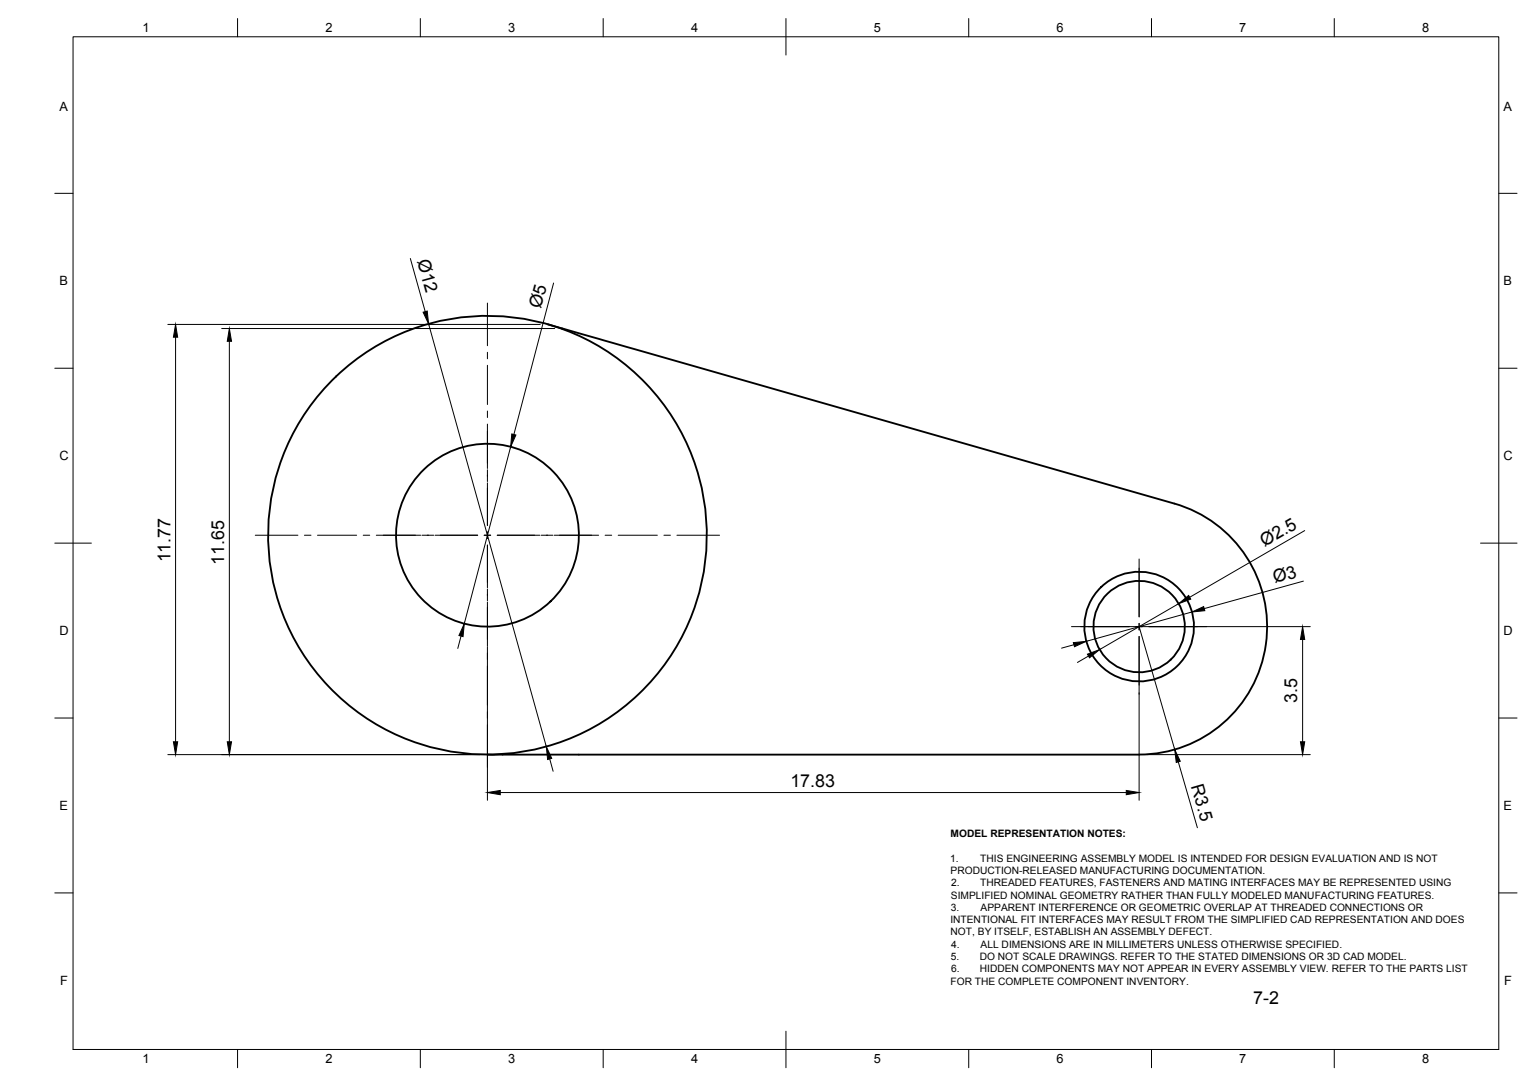
ISO-10303-21;
HEADER;
/* Generated by software containing ST-Developer
 * from STEP Tools, Inc. (www.steptools.com) 
 */

FILE_DESCRIPTION(
/* description */ (''),
/* implementation_level */ '2;1');

FILE_NAME(
/* name */ '7-2.step',
/* time_stamp */ '2026-10-06T01:16:10-07:00',
/* author */ (''),
/* organization */ (''),
/* preprocessor_version */ 'ST-DEVELOPER v20.2',
/* originating_system */ 'Autodesk Translation Framework v15.15.0.0',
/* authorisation */ '');

FILE_SCHEMA (('AUTOMOTIVE_DESIGN { 1 0 10303 214 3 1 1 }'));
ENDSEC;

DATA;
#10=MECHANICAL_DESIGN_GEOMETRIC_PRESENTATION_REPRESENTATION('',(#307,#308),#17113);
#107=ELLIPSE('',#6627,1.26223360526973,1.25);
#108=ELLIPSE('',#6640,1.26223360526973,1.25);
#135=TOROIDAL_SURFACE('',#6625,6.5,0.5);
#136=TOROIDAL_SURFACE('',#6631,5.7,0.3);
#137=TOROIDAL_SURFACE('',#6636,3.2,0.3);
#176=B_SPLINE_CURVE_WITH_KNOTS('',3,(#10699,#10700,#10701,#10702,#10703,
#10704,#10705,#10706,#10707,#10708),.UNSPECIFIED.,.F.,.F.,(4,2,2,2,4),(-0.377880095159423,
-0.330643519967439,-0.283406944775455,-0.236173496177583,-0.188940047579712),
 .UNSPECIFIED.);
#177=B_SPLINE_CURVE_WITH_KNOTS('',3,(#10712,#10713,#10714,#10715,#10716,
#10717,#10718,#10719,#10720,#10721),.UNSPECIFIED.,.F.,.F.,(4,2,2,2,4),(0.188940047579712,
0.236173496177583,0.283406944775455,0.330643519967439,0.377880095159423),
 .UNSPECIFIED.);
#178=B_SPLINE_CURVE_WITH_KNOTS('',3,(#10723,#10724,#10725,#10726,#10727,
#10728,#10729,#10730,#10731,#10732,#10733,#10734,#10735,#10736,#10737,#10738,
#10739,#10740,#10741,#10742,#10743,#10744,#10745),.UNSPECIFIED.,.F.,.F.,
(4,2,2,2,2,2,3,2,2,2,4),(-0.276474823920439,-0.236173496177583,-0.188940047579712,
-0.14170659898184,-0.0944731503839682,-0.0472365751919841,0.,0.0472365751919841,
0.0944731503839681,0.14170659898184,0.188940047579712),.UNSPECIFIED.);
#179=B_SPLINE_CURVE_WITH_KNOTS('',3,(#10752,#10753,#10754,#10755,#10756,
#10757,#10758,#10759,#10760,#10761,#10762,#10763,#10764,#10765,#10766,#10767,
#10768,#10769,#10770),.UNSPECIFIED.,.F.,.F.,(4,2,2,2,3,2,2,2,4),(-0.188940047579712,
-0.14170659898184,-0.0944731503839681,-0.0472365751919841,0.,0.0472365751919841,
0.0944731503839682,0.14170659898184,0.188940047579712),.UNSPECIFIED.);
#180=B_SPLINE_CURVE_WITH_KNOTS('',3,(#10799,#10800,#10801,#10802),
 .UNSPECIFIED.,.F.,.F.,(4,4),(0.0419009061515246,0.24114214195851),
 .UNSPECIFIED.);
#181=B_SPLINE_CURVE_WITH_KNOTS('',3,(#10803,#10804,#10805,#10806,#10807,
#10808),.UNSPECIFIED.,.F.,.F.,(4,2,4),(-0.160890299009028,-0.155410119436095,
-0.148763314259543),.UNSPECIFIED.);
#182=B_SPLINE_CURVE_WITH_KNOTS('',3,(#10810,#10811,#10812,#10813,#10814,
#10815),.UNSPECIFIED.,.F.,.F.,(4,2,4),(-0.173042755318085,-0.172254926856018,
-0.160890299013474),.UNSPECIFIED.);
#183=B_SPLINE_CURVE_WITH_KNOTS('',3,(#10816,#10817,#10818,#10819),
 .UNSPECIFIED.,.F.,.F.,(4,4),(0.488884303449535,0.688125539256493),
 .UNSPECIFIED.);
#184=B_SPLINE_CURVE_WITH_KNOTS('',3,(#10845,#10846,#10847,#10848,#10849,
#10850),.UNSPECIFIED.,.F.,.F.,(4,2,4),(0.188940047579712,0.236173496177584,
0.276474823920109),.UNSPECIFIED.);
#185=B_SPLINE_CURVE_WITH_KNOTS('',3,(#10854,#10855,#10856,#10857,#10858,
#10859,#10860,#10861,#10862,#10863,#10864,#10865,#10866,#10867,#10868,#10869,
#10870,#10871),.UNSPECIFIED.,.F.,.F.,(4,2,2,2,2,2,2,2,4),(0.192195276051885,
0.240178513967644,0.288161751883402,0.336276151993586,0.38439055210377,
0.432504952213954,0.480619352324138,0.528602590239897,0.576585828155655),
 .UNSPECIFIED.);
#186=B_SPLINE_CURVE_WITH_KNOTS('',3,(#10872,#10873,#10874,#10875,#10876,
#10877,#10878,#10879,#10880,#10881,#10882,#10883,#10884,#10885,#10886,#10887,
#10888,#10889,#10890),.UNSPECIFIED.,.F.,.F.,(4,2,2,2,3,2,2,2,4),(-0.192195276051885,
-0.144212038136127,-0.0962288002203683,-0.0481144001101841,1.11022302462516E-16,
0.0481144001101843,0.0962288002203684,0.144212038136127,0.192195276051885),
 .UNSPECIFIED.);
#187=B_SPLINE_CURVE_WITH_KNOTS('',3,(#10894,#10895,#10896,#10897,#10898,
#10899,#10900,#10901,#10902,#10903,#10904,#10905,#10906,#10907,#10908,#10909,
#10910,#10911,#10912),.UNSPECIFIED.,.F.,.F.,(4,2,2,2,3,2,2,2,4),(-0.192195276051885,
-0.144212038136127,-0.0962288002203683,-0.0481144001101841,0.,0.0481144001101841,
0.0962288002203683,0.144212038136127,0.192195276051885),.UNSPECIFIED.);
#188=B_SPLINE_CURVE_WITH_KNOTS('',3,(#10913,#10914,#10915,#10916,#10917,
#10918,#10919,#10920,#10921,#10922,#10923,#10924,#10925,#10926,#10927,#10928,
#10929,#10930),.UNSPECIFIED.,.F.,.F.,(4,2,2,2,2,2,2,2,4),(0.192195276051885,
0.240178513967643,0.288161751883402,0.336276151993586,0.38439055210377,
0.432504952213954,0.480619352324138,0.528602590239897,0.576585828155655),
 .UNSPECIFIED.);
#227=OPEN_SHELL('',(#5864,#5865));
#245=SHELL_BASED_SURFACE_MODEL('Body2',(#227));
#269=SHAPE_REPRESENTATION_RELATIONSHIP('SRR','None',#17193,#285);
#285=ADVANCED_BREP_SHAPE_REPRESENTATION('',(#335),#17100);
#307=STYLED_ITEM('',(#17298),#335);
#308=STYLED_ITEM('',(#17298),#245);
#335=MANIFOLD_SOLID_BREP('Body1',#6021);
#431=CYLINDRICAL_SURFACE('',#6611,6.);
#432=CYLINDRICAL_SURFACE('',#6620,1.25);
#433=CYLINDRICAL_SURFACE('',#6628,0.3);
#434=CYLINDRICAL_SURFACE('',#6634,0.3);
#435=CYLINDRICAL_SURFACE('',#6638,3.5);
#436=CYLINDRICAL_SURFACE('',#6641,1.25);
#437=CYLINDRICAL_SURFACE('',#6642,1.25);
#438=CYLINDRICAL_SURFACE('',#6643,6.);
#439=CYLINDRICAL_SURFACE('',#6644,2.5);
#440=CYLINDRICAL_SURFACE('',#6647,1.5);
#577=FACE_BOUND('',#1634,.T.);
#578=FACE_BOUND('',#1635,.T.);
#579=FACE_BOUND('',#1638,.T.);
#580=FACE_BOUND('',#1651,.T.);
#581=FACE_BOUND('',#1653,.T.);
#582=FACE_BOUND('',#1656,.T.);
#836=CIRCLE('',#6612,6.);
#837=CIRCLE('',#6613,6.);
#838=CIRCLE('',#6614,6.);
#839=CIRCLE('',#6616,5.7);
#840=CIRCLE('',#6617,3.2);
#841=CIRCLE('',#6618,2.5);
#842=CIRCLE('',#6619,1.25);
#843=CIRCLE('',#6621,1.25);
#844=CIRCLE('',#6623,6.5);
#845=CIRCLE('',#6624,3.5);
#846=CIRCLE('',#6629,0.3);
#847=CIRCLE('',#6630,0.3);
#848=CIRCLE('',#6632,6.);
#849=CIRCLE('',#6633,0.3);
#850=CIRCLE('',#6635,0.3);
#851=CIRCLE('',#6637,3.5);
#852=CIRCLE('',#6645,2.5);
#853=CIRCLE('',#6648,1.5);
#854=CIRCLE('',#6649,1.5);
#855=CIRCLE('',#6651,1.25);
#1199=FACE_OUTER_BOUND('',#1632,.T.);
#1200=FACE_OUTER_BOUND('',#1633,.T.);
#1201=FACE_OUTER_BOUND('',#1636,.T.);
#1202=FACE_OUTER_BOUND('',#1637,.T.);
#1203=FACE_OUTER_BOUND('',#1639,.T.);
#1204=FACE_OUTER_BOUND('',#1640,.T.);
#1205=FACE_OUTER_BOUND('',#1641,.T.);
#1206=FACE_OUTER_BOUND('',#1642,.T.);
#1207=FACE_OUTER_BOUND('',#1643,.T.);
#1208=FACE_OUTER_BOUND('',#1644,.T.);
#1209=FACE_OUTER_BOUND('',#1645,.T.);
#1210=FACE_OUTER_BOUND('',#1646,.T.);
#1211=FACE_OUTER_BOUND('',#1647,.T.);
#1212=FACE_OUTER_BOUND('',#1648,.T.);
#1213=FACE_OUTER_BOUND('',#1649,.T.);
#1214=FACE_OUTER_BOUND('',#1650,.T.);
#1215=FACE_OUTER_BOUND('',#1652,.T.);
#1216=FACE_OUTER_BOUND('',#1654,.T.);
#1217=FACE_OUTER_BOUND('',#1655,.T.);
#1632=EDGE_LOOP('',(#4788,#4789,#4790,#4791,#4792,#4793,#4794,#4795,#4796,
#4797,#4798));
#1633=EDGE_LOOP('',(#4799,#4800,#4801,#4802));
#1634=EDGE_LOOP('',(#4803));
#1635=EDGE_LOOP('',(#4804));
#1636=EDGE_LOOP('',(#4805,#4806,#4807,#4808));
#1637=EDGE_LOOP('',(#4809,#4810,#4811,#4812));
#1638=EDGE_LOOP('',(#4813));
#1639=EDGE_LOOP('',(#4814,#4815,#4816,#4817,#4818,#4819));
#1640=EDGE_LOOP('',(#4820,#4821,#4822,#4823,#4824,#4825));
#1641=EDGE_LOOP('',(#4826,#4827,#4828,#4829));
#1642=EDGE_LOOP('',(#4830,#4831,#4832,#4833,#4834));
#1643=EDGE_LOOP('',(#4835,#4836,#4837,#4838));
#1644=EDGE_LOOP('',(#4839,#4840,#4841,#4842));
#1645=EDGE_LOOP('',(#4843,#4844,#4845,#4846));
#1646=EDGE_LOOP('',(#4847,#4848,#4849,#4850,#4851,#4852));
#1647=EDGE_LOOP('',(#4853,#4854,#4855,#4856,#4857,#4858,#4859,#4860,#4861));
#1648=EDGE_LOOP('',(#4862,#4863,#4864,#4865,#4866,#4867,#4868,#4869));
#1649=EDGE_LOOP('',(#4870,#4871,#4872,#4873));
#1650=EDGE_LOOP('',(#4874,#4875,#4876,#4877,#4878,#4879,#4880,#4881));
#1651=EDGE_LOOP('',(#4882,#4883));
#1652=EDGE_LOOP('',(#4884));
#1653=EDGE_LOOP('',(#4885));
#1654=EDGE_LOOP('',(#4886,#4887,#4888,#4889));
#1655=EDGE_LOOP('',(#4890));
#1656=EDGE_LOOP('',(#4891));
#2070=LINE('',#10697,#2431);
#2071=LINE('',#10747,#2432);
#2072=LINE('',#10751,#2433);
#2073=LINE('',#10776,#2434);
#2074=LINE('',#10779,#2435);
#2075=LINE('',#10786,#2436);
#2076=LINE('',#10793,#2437);
#2077=LINE('',#10796,#2438);
#2078=LINE('',#10823,#2439);
#2079=LINE('',#10824,#2440);
#2080=LINE('',#10827,#2441);
#2081=LINE('',#10836,#2442);
#2082=LINE('',#10841,#2443);
#2083=LINE('',#10852,#2444);
#2084=LINE('',#10931,#2445);
#2085=LINE('',#10934,#2446);
#2086=LINE('',#10936,#2447);
#2087=LINE('',#10943,#2448);
#2431=VECTOR('',#7996,6.);
#2432=VECTOR('',#7999,3.268305009375);
#2433=VECTOR('',#8002,6.);
#2434=VECTOR('',#8007,17.82554346998);
#2435=VECTOR('',#8010,17.8255434699797);
#2436=VECTOR('',#8017,1.25);
#2437=VECTOR('',#8024,15.3255434699798);
#2438=VECTOR('',#8027,15.3255434699798);
#2439=VECTOR('',#8032,17.8255434887197);
#2440=VECTOR('',#8033,3.7);
#2441=VECTOR('',#8036,3.268305009375);
#2442=VECTOR('',#8051,17.8255434620497);
#2443=VECTOR('',#8060,3.7);
#2444=VECTOR('',#8067,1.25);
#2445=VECTOR('',#8070,1.25);
#2446=VECTOR('',#8075,2.5);
#2447=VECTOR('',#8076,2.5);
#2448=VECTOR('',#8085,1.5);
#2858=VERTEX_POINT('',#10694);
#2859=VERTEX_POINT('',#10696);
#2860=VERTEX_POINT('',#10698);
#2861=VERTEX_POINT('',#10709);
#2862=VERTEX_POINT('',#10711);
#2863=VERTEX_POINT('',#10722);
#2864=VERTEX_POINT('',#10746);
#2865=VERTEX_POINT('',#10748);
#2866=VERTEX_POINT('',#10750);
#2867=VERTEX_POINT('',#10772);
#2868=VERTEX_POINT('',#10773);
#2869=VERTEX_POINT('',#10775);
#2870=VERTEX_POINT('',#10777);
#2871=VERTEX_POINT('',#10780);
#2872=VERTEX_POINT('',#10782);
#2873=VERTEX_POINT('',#10785);
#2874=VERTEX_POINT('',#10789);
#2875=VERTEX_POINT('',#10790);
#2876=VERTEX_POINT('',#10792);
#2877=VERTEX_POINT('',#10794);
#2878=VERTEX_POINT('',#10798);
#2879=VERTEX_POINT('',#10809);
#2880=VERTEX_POINT('',#10821);
#2881=VERTEX_POINT('',#10822);
#2882=VERTEX_POINT('',#10825);
#2883=VERTEX_POINT('',#10835);
#2884=VERTEX_POINT('',#10851);
#2885=VERTEX_POINT('',#10853);
#2886=VERTEX_POINT('',#10892);
#2887=VERTEX_POINT('',#10893);
#2888=VERTEX_POINT('',#10935);
#2889=VERTEX_POINT('',#10940);
#2890=VERTEX_POINT('',#10942);
#2891=VERTEX_POINT('',#10946);
#3546=EDGE_CURVE('',#2858,#2858,#836,.T.);
#3547=EDGE_CURVE('',#2858,#2859,#2070,.T.);
#3548=EDGE_CURVE('',#2859,#2860,#176,.F.);
#3549=EDGE_CURVE('',#2860,#2861,#837,.T.);
#3550=EDGE_CURVE('',#2861,#2862,#177,.F.);
#3551=EDGE_CURVE('',#2862,#2863,#178,.F.);
#3552=EDGE_CURVE('',#2864,#2863,#2071,.T.);
#3553=EDGE_CURVE('',#2865,#2864,#838,.T.);
#3554=EDGE_CURVE('',#2866,#2865,#2072,.T.);
#3555=EDGE_CURVE('',#2866,#2859,#179,.F.);
#3556=EDGE_CURVE('',#2867,#2868,#839,.T.);
#3557=EDGE_CURVE('',#2868,#2869,#2073,.T.);
#3558=EDGE_CURVE('',#2869,#2870,#840,.T.);
#3559=EDGE_CURVE('',#2870,#2867,#2074,.T.);
#3560=EDGE_CURVE('',#2871,#2871,#841,.T.);
#3561=EDGE_CURVE('',#2872,#2872,#842,.T.);
#3562=EDGE_CURVE('',#2872,#2873,#2075,.T.);
#3563=EDGE_CURVE('',#2873,#2873,#843,.T.);
#3564=EDGE_CURVE('',#2874,#2875,#844,.T.);
#3565=EDGE_CURVE('',#2874,#2876,#2076,.T.);
#3566=EDGE_CURVE('',#2876,#2877,#845,.T.);
#3567=EDGE_CURVE('',#2877,#2875,#2077,.T.);
#3568=EDGE_CURVE('',#2878,#2875,#180,.T.);
#3569=EDGE_CURVE('',#2861,#2878,#181,.T.);
#3570=EDGE_CURVE('',#2879,#2860,#182,.T.);
#3571=EDGE_CURVE('',#2874,#2879,#183,.T.);
#3572=EDGE_CURVE('',#2880,#2881,#2078,.T.);
#3573=EDGE_CURVE('',#2880,#2876,#2079,.T.);
#3574=EDGE_CURVE('',#2879,#2882,#107,.T.);
#3575=EDGE_CURVE('',#2881,#2882,#2080,.T.);
#3576=EDGE_CURVE('',#2870,#2880,#846,.T.);
#3577=EDGE_CURVE('',#2867,#2881,#847,.T.);
#3578=EDGE_CURVE('',#2881,#2865,#848,.T.);
#3579=EDGE_CURVE('',#2868,#2864,#849,.T.);
#3580=EDGE_CURVE('',#2864,#2883,#2081,.T.);
#3581=EDGE_CURVE('',#2869,#2883,#850,.T.);
#3582=EDGE_CURVE('',#2883,#2880,#851,.T.);
#3583=EDGE_CURVE('',#2883,#2877,#2082,.T.);
#3584=EDGE_CURVE('',#2878,#2863,#108,.T.);
#3585=EDGE_CURVE('',#2882,#2866,#184,.F.);
#3586=EDGE_CURVE('',#2859,#2884,#2083,.T.);
#3587=EDGE_CURVE('',#2885,#2884,#185,.T.);
#3588=EDGE_CURVE('',#2884,#2885,#186,.T.);
#3589=EDGE_CURVE('',#2886,#2887,#187,.T.);
#3590=EDGE_CURVE('',#2887,#2886,#188,.T.);
#3591=EDGE_CURVE('',#2887,#2862,#2084,.T.);
#3592=EDGE_CURVE('',#2871,#2885,#2085,.T.);
#3593=EDGE_CURVE('',#2884,#2888,#2086,.T.);
#3594=EDGE_CURVE('',#2888,#2888,#852,.T.);
#3595=EDGE_CURVE('',#2889,#2889,#853,.T.);
#3596=EDGE_CURVE('',#2889,#2890,#2087,.T.);
#3597=EDGE_CURVE('',#2890,#2890,#854,.T.);
#3598=EDGE_CURVE('',#2891,#2891,#855,.T.);
#4788=ORIENTED_EDGE('',*,*,#3546,.F.);
#4789=ORIENTED_EDGE('',*,*,#3547,.T.);
#4790=ORIENTED_EDGE('',*,*,#3548,.T.);
#4791=ORIENTED_EDGE('',*,*,#3549,.T.);
#4792=ORIENTED_EDGE('',*,*,#3550,.T.);
#4793=ORIENTED_EDGE('',*,*,#3551,.T.);
#4794=ORIENTED_EDGE('',*,*,#3552,.F.);
#4795=ORIENTED_EDGE('',*,*,#3553,.F.);
#4796=ORIENTED_EDGE('',*,*,#3554,.F.);
#4797=ORIENTED_EDGE('',*,*,#3555,.T.);
#4798=ORIENTED_EDGE('',*,*,#3547,.F.);
#4799=ORIENTED_EDGE('',*,*,#3556,.T.);
#4800=ORIENTED_EDGE('',*,*,#3557,.T.);
#4801=ORIENTED_EDGE('',*,*,#3558,.T.);
#4802=ORIENTED_EDGE('',*,*,#3559,.T.);
#4803=ORIENTED_EDGE('',*,*,#3560,.F.);
#4804=ORIENTED_EDGE('',*,*,#3561,.F.);
#4805=ORIENTED_EDGE('',*,*,#3561,.T.);
#4806=ORIENTED_EDGE('',*,*,#3562,.T.);
#4807=ORIENTED_EDGE('',*,*,#3563,.F.);
#4808=ORIENTED_EDGE('',*,*,#3562,.F.);
#4809=ORIENTED_EDGE('',*,*,#3564,.F.);
#4810=ORIENTED_EDGE('',*,*,#3565,.T.);
#4811=ORIENTED_EDGE('',*,*,#3566,.T.);
#4812=ORIENTED_EDGE('',*,*,#3567,.T.);
#4813=ORIENTED_EDGE('',*,*,#3563,.T.);
#4814=ORIENTED_EDGE('',*,*,#3564,.T.);
#4815=ORIENTED_EDGE('',*,*,#3568,.F.);
#4816=ORIENTED_EDGE('',*,*,#3569,.F.);
#4817=ORIENTED_EDGE('',*,*,#3549,.F.);
#4818=ORIENTED_EDGE('',*,*,#3570,.F.);
#4819=ORIENTED_EDGE('',*,*,#3571,.F.);
#4820=ORIENTED_EDGE('',*,*,#3572,.F.);
#4821=ORIENTED_EDGE('',*,*,#3573,.T.);
#4822=ORIENTED_EDGE('',*,*,#3565,.F.);
#4823=ORIENTED_EDGE('',*,*,#3571,.T.);
#4824=ORIENTED_EDGE('',*,*,#3574,.T.);
#4825=ORIENTED_EDGE('',*,*,#3575,.F.);
#4826=ORIENTED_EDGE('',*,*,#3559,.F.);
#4827=ORIENTED_EDGE('',*,*,#3576,.T.);
#4828=ORIENTED_EDGE('',*,*,#3572,.T.);
#4829=ORIENTED_EDGE('',*,*,#3577,.F.);
#4830=ORIENTED_EDGE('',*,*,#3556,.F.);
#4831=ORIENTED_EDGE('',*,*,#3577,.T.);
#4832=ORIENTED_EDGE('',*,*,#3578,.T.);
#4833=ORIENTED_EDGE('',*,*,#3553,.T.);
#4834=ORIENTED_EDGE('',*,*,#3579,.F.);
#4835=ORIENTED_EDGE('',*,*,#3557,.F.);
#4836=ORIENTED_EDGE('',*,*,#3579,.T.);
#4837=ORIENTED_EDGE('',*,*,#3580,.T.);
#4838=ORIENTED_EDGE('',*,*,#3581,.F.);
#4839=ORIENTED_EDGE('',*,*,#3558,.F.);
#4840=ORIENTED_EDGE('',*,*,#3581,.T.);
#4841=ORIENTED_EDGE('',*,*,#3582,.T.);
#4842=ORIENTED_EDGE('',*,*,#3576,.F.);
#4843=ORIENTED_EDGE('',*,*,#3582,.F.);
#4844=ORIENTED_EDGE('',*,*,#3583,.T.);
#4845=ORIENTED_EDGE('',*,*,#3566,.F.);
#4846=ORIENTED_EDGE('',*,*,#3573,.F.);
#4847=ORIENTED_EDGE('',*,*,#3580,.F.);
#4848=ORIENTED_EDGE('',*,*,#3552,.T.);
#4849=ORIENTED_EDGE('',*,*,#3584,.F.);
#4850=ORIENTED_EDGE('',*,*,#3568,.T.);
#4851=ORIENTED_EDGE('',*,*,#3567,.F.);
#4852=ORIENTED_EDGE('',*,*,#3583,.F.);
#4853=ORIENTED_EDGE('',*,*,#3585,.F.);
#4854=ORIENTED_EDGE('',*,*,#3574,.F.);
#4855=ORIENTED_EDGE('',*,*,#3570,.T.);
#4856=ORIENTED_EDGE('',*,*,#3548,.F.);
#4857=ORIENTED_EDGE('',*,*,#3586,.T.);
#4858=ORIENTED_EDGE('',*,*,#3587,.F.);
#4859=ORIENTED_EDGE('',*,*,#3588,.F.);
#4860=ORIENTED_EDGE('',*,*,#3586,.F.);
#4861=ORIENTED_EDGE('',*,*,#3555,.F.);
#4862=ORIENTED_EDGE('',*,*,#3589,.F.);
#4863=ORIENTED_EDGE('',*,*,#3590,.F.);
#4864=ORIENTED_EDGE('',*,*,#3591,.T.);
#4865=ORIENTED_EDGE('',*,*,#3550,.F.);
#4866=ORIENTED_EDGE('',*,*,#3569,.T.);
#4867=ORIENTED_EDGE('',*,*,#3584,.T.);
#4868=ORIENTED_EDGE('',*,*,#3551,.F.);
#4869=ORIENTED_EDGE('',*,*,#3591,.F.);
#4870=ORIENTED_EDGE('',*,*,#3554,.T.);
#4871=ORIENTED_EDGE('',*,*,#3578,.F.);
#4872=ORIENTED_EDGE('',*,*,#3575,.T.);
#4873=ORIENTED_EDGE('',*,*,#3585,.T.);
#4874=ORIENTED_EDGE('',*,*,#3560,.T.);
#4875=ORIENTED_EDGE('',*,*,#3592,.T.);
#4876=ORIENTED_EDGE('',*,*,#3587,.T.);
#4877=ORIENTED_EDGE('',*,*,#3593,.T.);
#4878=ORIENTED_EDGE('',*,*,#3594,.F.);
#4879=ORIENTED_EDGE('',*,*,#3593,.F.);
#4880=ORIENTED_EDGE('',*,*,#3588,.T.);
#4881=ORIENTED_EDGE('',*,*,#3592,.F.);
#4882=ORIENTED_EDGE('',*,*,#3589,.T.);
#4883=ORIENTED_EDGE('',*,*,#3590,.T.);
#4884=ORIENTED_EDGE('',*,*,#3546,.T.);
#4885=ORIENTED_EDGE('',*,*,#3594,.T.);
#4886=ORIENTED_EDGE('',*,*,#3595,.F.);
#4887=ORIENTED_EDGE('',*,*,#3596,.T.);
#4888=ORIENTED_EDGE('',*,*,#3597,.T.);
#4889=ORIENTED_EDGE('',*,*,#3596,.F.);
#4890=ORIENTED_EDGE('',*,*,#3597,.F.);
#4891=ORIENTED_EDGE('',*,*,#3598,.F.);
#5577=PLANE('',#6615);
#5578=PLANE('',#6622);
#5579=PLANE('',#6626);
#5580=PLANE('',#6639);
#5581=PLANE('',#6646);
#5582=PLANE('',#6650);
#5847=ADVANCED_FACE('',(#1199),#431,.T.);
#5848=ADVANCED_FACE('',(#1200,#577,#578),#5577,.F.);
#5849=ADVANCED_FACE('',(#1201),#432,.F.);
#5850=ADVANCED_FACE('',(#1202,#579),#5578,.T.);
#5851=ADVANCED_FACE('',(#1203),#135,.F.);
#5852=ADVANCED_FACE('',(#1204),#5579,.T.);
#5853=ADVANCED_FACE('',(#1205),#433,.T.);
#5854=ADVANCED_FACE('',(#1206),#136,.T.);
#5855=ADVANCED_FACE('',(#1207),#434,.T.);
#5856=ADVANCED_FACE('',(#1208),#137,.T.);
#5857=ADVANCED_FACE('',(#1209),#435,.T.);
#5858=ADVANCED_FACE('',(#1210),#5580,.T.);
#5859=ADVANCED_FACE('',(#1211),#436,.F.);
#5860=ADVANCED_FACE('',(#1212),#437,.F.);
#5861=ADVANCED_FACE('',(#1213),#438,.T.);
#5862=ADVANCED_FACE('',(#1214,#580),#439,.F.);
#5863=ADVANCED_FACE('',(#1215,#581),#5581,.T.);
#5864=ADVANCED_FACE('',(#1216),#440,.T.);
#5865=ADVANCED_FACE('',(#1217,#582),#5582,.F.);
#6021=CLOSED_SHELL('',(#5847,#5848,#5849,#5850,#5851,#5852,#5853,#5854,
#5855,#5856,#5857,#5858,#5859,#5860,#5861,#5862,#5863));
#6610=AXIS2_PLACEMENT_3D('',#10692,#7990,#7991);
#6611=AXIS2_PLACEMENT_3D('',#10693,#7992,#7993);
#6612=AXIS2_PLACEMENT_3D('',#10695,#7994,#7995);
#6613=AXIS2_PLACEMENT_3D('',#10710,#7997,#7998);
#6614=AXIS2_PLACEMENT_3D('',#10749,#8000,#8001);
#6615=AXIS2_PLACEMENT_3D('',#10771,#8003,#8004);
#6616=AXIS2_PLACEMENT_3D('',#10774,#8005,#8006);
#6617=AXIS2_PLACEMENT_3D('',#10778,#8008,#8009);
#6618=AXIS2_PLACEMENT_3D('',#10781,#8011,#8012);
#6619=AXIS2_PLACEMENT_3D('',#10783,#8013,#8014);
#6620=AXIS2_PLACEMENT_3D('',#10784,#8015,#8016);
#6621=AXIS2_PLACEMENT_3D('',#10787,#8018,#8019);
#6622=AXIS2_PLACEMENT_3D('',#10788,#8020,#8021);
#6623=AXIS2_PLACEMENT_3D('',#10791,#8022,#8023);
#6624=AXIS2_PLACEMENT_3D('',#10795,#8025,#8026);
#6625=AXIS2_PLACEMENT_3D('',#10797,#8028,#8029);
#6626=AXIS2_PLACEMENT_3D('',#10820,#8030,#8031);
#6627=AXIS2_PLACEMENT_3D('',#10826,#8034,#8035);
#6628=AXIS2_PLACEMENT_3D('',#10828,#8037,#8038);
#6629=AXIS2_PLACEMENT_3D('',#10829,#8039,#8040);
#6630=AXIS2_PLACEMENT_3D('',#10830,#8041,#8042);
#6631=AXIS2_PLACEMENT_3D('',#10831,#8043,#8044);
#6632=AXIS2_PLACEMENT_3D('',#10832,#8045,#8046);
#6633=AXIS2_PLACEMENT_3D('',#10833,#8047,#8048);
#6634=AXIS2_PLACEMENT_3D('',#10834,#8049,#8050);
#6635=AXIS2_PLACEMENT_3D('',#10837,#8052,#8053);
#6636=AXIS2_PLACEMENT_3D('',#10838,#8054,#8055);
#6637=AXIS2_PLACEMENT_3D('',#10839,#8056,#8057);
#6638=AXIS2_PLACEMENT_3D('',#10840,#8058,#8059);
#6639=AXIS2_PLACEMENT_3D('',#10842,#8061,#8062);
#6640=AXIS2_PLACEMENT_3D('',#10843,#8063,#8064);
#6641=AXIS2_PLACEMENT_3D('',#10844,#8065,#8066);
#6642=AXIS2_PLACEMENT_3D('',#10891,#8068,#8069);
#6643=AXIS2_PLACEMENT_3D('',#10932,#8071,#8072);
#6644=AXIS2_PLACEMENT_3D('',#10933,#8073,#8074);
#6645=AXIS2_PLACEMENT_3D('',#10937,#8077,#8078);
#6646=AXIS2_PLACEMENT_3D('',#10938,#8079,#8080);
#6647=AXIS2_PLACEMENT_3D('',#10939,#8081,#8082);
#6648=AXIS2_PLACEMENT_3D('',#10941,#8083,#8084);
#6649=AXIS2_PLACEMENT_3D('',#10944,#8086,#8087);
#6650=AXIS2_PLACEMENT_3D('',#10945,#8088,#8089);
#6651=AXIS2_PLACEMENT_3D('',#10947,#8090,#8091);
#7990=DIRECTION('axis',(0.,0.,1.));
#7991=DIRECTION('refdir',(1.,0.,0.));
#7992=DIRECTION('center_axis',(0.,0.,1.));
#7993=DIRECTION('ref_axis',(1.,0.,0.));
#7994=DIRECTION('center_axis',(0.,0.,1.));
#7995=DIRECTION('ref_axis',(-1.,0.,0.));
#7996=DIRECTION('',(0.,0.,-1.));
#7997=DIRECTION('center_axis',(0.,0.,1.));
#7998=DIRECTION('ref_axis',(-0.978057882858799,-0.2083333333333,0.));
#7999=DIRECTION('',(-3.360919818376E-10,-2.396404589967E-9,1.));
#8000=DIRECTION('center_axis',(0.,0.,-1.));
#8001=DIRECTION('ref_axis',(-0.990307970554214,-0.138888888888902,0.));
#8002=DIRECTION('',(0.,0.,-1.));
#8003=DIRECTION('center_axis',(0.,0.,1.));
#8004=DIRECTION('ref_axis',(1.,0.,0.));
#8005=DIRECTION('center_axis',(0.,0.,-1.));
#8006=DIRECTION('ref_axis',(-0.990307970554214,-0.138888888888902,0.));
#8007=DIRECTION('',(-0.138888888889,-0.9903079705542,0.));
#8008=DIRECTION('center_axis',(0.,0.,-1.));
#8009=DIRECTION('ref_axis',(0.990307970554214,-0.138888888888902,0.));
#8010=DIRECTION('',(-0.138888888888902,0.990307970554214,0.));
#8011=DIRECTION('center_axis',(0.,0.,-1.));
#8012=DIRECTION('ref_axis',(1.,0.,0.));
#8013=DIRECTION('center_axis',(0.,0.,-1.));
#8014=DIRECTION('ref_axis',(1.,0.,0.));
#8015=DIRECTION('center_axis',(0.,0.,1.));
#8016=DIRECTION('ref_axis',(1.,0.,0.));
#8017=DIRECTION('',(0.,0.,1.));
#8018=DIRECTION('center_axis',(0.,0.,-1.));
#8019=DIRECTION('ref_axis',(1.,0.,0.));
#8020=DIRECTION('center_axis',(0.,0.,1.));
#8021=DIRECTION('ref_axis',(1.,0.,0.));
#8022=DIRECTION('center_axis',(0.,0.,1.));
#8023=DIRECTION('ref_axis',(-0.860711630938934,-0.50909280918752,0.));
#8024=DIRECTION('',(0.138888888888902,-0.990307970554214,0.));
#8025=DIRECTION('center_axis',(0.,0.,1.));
#8026=DIRECTION('ref_axis',(-0.990307970554214,-0.138888888888902,0.));
#8027=DIRECTION('',(0.138888888888902,0.990307970554214,0.));
#8028=DIRECTION('center_axis',(0.,0.,1.));
#8029=DIRECTION('ref_axis',(1.16333808905522E-13,-1.,0.));
#8030=DIRECTION('center_axis',(-0.990307970554214,-0.138888888888902,0.));
#8031=DIRECTION('ref_axis',(0.138888888888902,-0.990307970554214,0.));
#8032=DIRECTION('',(-0.138888888888902,0.990307970554214,0.));
#8033=DIRECTION('',(-8.499803863751E-10,6.060543553496E-9,1.));
#8034=DIRECTION('center_axis',(0.990307970554214,0.138888888888902,0.));
#8035=DIRECTION('ref_axis',(-0.138888888888902,0.990307970554214,0.));
#8036=DIRECTION('',(-1.658618955119E-10,1.182636708731E-9,1.));
#8037=DIRECTION('center_axis',(-0.138888888888902,0.990307970554214,0.));
#8038=DIRECTION('ref_axis',(0.,0.,-1.));
#8039=DIRECTION('center_axis',(-0.138888888888902,0.990307970554214,0.));
#8040=DIRECTION('ref_axis',(0.,0.,-1.));
#8041=DIRECTION('center_axis',(-0.138888888888902,0.990307970554214,0.));
#8042=DIRECTION('ref_axis',(0.,0.,-1.));
#8043=DIRECTION('center_axis',(0.,0.,1.));
#8044=DIRECTION('ref_axis',(-8.09865507989116E-11,1.,0.));
#8045=DIRECTION('center_axis',(0.,0.,-1.));
#8046=DIRECTION('ref_axis',(-0.990307970554214,-0.138888888888902,0.));
#8047=DIRECTION('center_axis',(-0.138888888888902,-0.990307970554214,0.));
#8048=DIRECTION('ref_axis',(0.,0.,-1.));
#8049=DIRECTION('center_axis',(-0.138888888888902,-0.990307970554214,0.));
#8050=DIRECTION('ref_axis',(0.,0.,-1.));
#8051=DIRECTION('',(-0.138888888888902,-0.990307970554214,0.));
#8052=DIRECTION('center_axis',(-0.138888888888902,-0.990307970554214,0.));
#8053=DIRECTION('ref_axis',(0.,0.,-1.));
#8054=DIRECTION('center_axis',(0.,0.,1.));
#8055=DIRECTION('ref_axis',(0.997042419276589,-0.0768531987823992,0.));
#8056=DIRECTION('center_axis',(0.,0.,-1.));
#8057=DIRECTION('ref_axis',(0.990307970554214,-0.138888888888902,0.));
#8058=DIRECTION('center_axis',(0.,0.,1.));
#8059=DIRECTION('ref_axis',(1.,0.,0.));
#8060=DIRECTION('',(-5.942936233218E-10,-4.237442258943E-9,1.));
#8061=DIRECTION('center_axis',(0.990307970554214,-0.138888888888902,0.));
#8062=DIRECTION('ref_axis',(0.138888888888902,0.990307970554214,0.));
#8063=DIRECTION('center_axis',(0.990307970554214,-0.138888888888902,0.));
#8064=DIRECTION('ref_axis',(0.138888888888902,0.990307970554214,0.));
#8065=DIRECTION('center_axis',(1.,0.,0.));
#8066=DIRECTION('ref_axis',(0.,0.,-1.));
#8067=DIRECTION('',(1.,0.,0.));
#8068=DIRECTION('center_axis',(1.,0.,0.));
#8069=DIRECTION('ref_axis',(0.,0.,-1.));
#8070=DIRECTION('',(1.,0.,0.));
#8071=DIRECTION('center_axis',(0.,0.,1.));
#8072=DIRECTION('ref_axis',(1.,0.,0.));
#8073=DIRECTION('center_axis',(0.,0.,1.));
#8074=DIRECTION('ref_axis',(1.,0.,0.));
#8075=DIRECTION('',(0.,0.,1.));
#8076=DIRECTION('',(0.,0.,1.));
#8077=DIRECTION('center_axis',(0.,0.,-1.));
#8078=DIRECTION('ref_axis',(-1.,0.,0.));
#8079=DIRECTION('center_axis',(0.,0.,1.));
#8080=DIRECTION('ref_axis',(1.,0.,0.));
#8081=DIRECTION('center_axis',(0.,0.,1.));
#8082=DIRECTION('ref_axis',(1.,0.,0.));
#8083=DIRECTION('center_axis',(0.,0.,1.));
#8084=DIRECTION('ref_axis',(-1.,0.,0.));
#8085=DIRECTION('',(0.,0.,-1.));
#8086=DIRECTION('center_axis',(0.,0.,1.));
#8087=DIRECTION('ref_axis',(-1.,0.,0.));
#8088=DIRECTION('center_axis',(0.,0.,1.));
#8089=DIRECTION('ref_axis',(1.,0.,0.));
#8090=DIRECTION('center_axis',(0.,0.,-1.));
#8091=DIRECTION('ref_axis',(-1.,0.,0.));
#10692=CARTESIAN_POINT('',(0.,0.,0.));
#10693=CARTESIAN_POINT('Origin',(0.,18.,2.));
#10694=CARTESIAN_POINT('',(-6.,18.,5.));
#10695=CARTESIAN_POINT('Origin',(0.,18.,5.));
#10696=CARTESIAN_POINT('',(-6.,18.,3.75));
#10697=CARTESIAN_POINT('',(-6.,18.,2.));
#10698=CARTESIAN_POINT('',(-5.868347297153,16.75,2.5));
#10699=CARTESIAN_POINT('Ctrl Pts',(-5.86834729715275,16.75,2.5));
#10700=CARTESIAN_POINT('Ctrl Pts',(-5.86834729715275,16.75,2.65745525063995));
#10701=CARTESIAN_POINT('Ctrl Pts',(-5.87534197873269,16.7815621590215,2.82507913768158));
#10702=CARTESIAN_POINT('Ctrl Pts',(-5.90038488226116,16.9092698316582,3.13290995658393));
#10703=CARTESIAN_POINT('Ctrl Pts',(-5.91804743154611,17.0053912037911,3.27315815675743));
#10704=CARTESIAN_POINT('Ctrl Pts',(-5.9510289473619,17.2268345143215,3.49460146728784));
#10705=CARTESIAN_POINT('Ctrl Pts',(-5.96852269967858,17.3670858177603,3.59072857638709));
#10706=CARTESIAN_POINT('Ctrl Pts',(-5.99317707212167,17.6749274551324,3.71844041497889));
#10707=CARTESIAN_POINT('Ctrl Pts',(-6.,17.8425551713404,3.75));
#10708=CARTESIAN_POINT('Ctrl Pts',(-6.,18.,3.75));
#10709=CARTESIAN_POINT('',(5.868347297153,16.75,2.5));
#10710=CARTESIAN_POINT('Origin',(0.,18.,2.5));
#10711=CARTESIAN_POINT('',(6.,18.,3.75));
#10712=CARTESIAN_POINT('Ctrl Pts',(6.,18.,3.75));
#10713=CARTESIAN_POINT('Ctrl Pts',(6.,17.8425551713404,3.75));
#10714=CARTESIAN_POINT('Ctrl Pts',(5.99317707212168,17.6749274551324,3.71844041497889));
#10715=CARTESIAN_POINT('Ctrl Pts',(5.96852269967858,17.3670858177603,3.59072857638709));
#10716=CARTESIAN_POINT('Ctrl Pts',(5.9510289473619,17.2268345143215,3.49460146728784));
#10717=CARTESIAN_POINT('Ctrl Pts',(5.91804743154611,17.0053912037911,3.27315815675743));
#10718=CARTESIAN_POINT('Ctrl Pts',(5.90038488226116,16.9092698316582,3.13290995658393));
#10719=CARTESIAN_POINT('Ctrl Pts',(5.87534197873269,16.7815621590215,2.82507913768158));
#10720=CARTESIAN_POINT('Ctrl Pts',(5.86834729715275,16.75,2.65745525063995));
#10721=CARTESIAN_POINT('Ctrl Pts',(5.86834729715275,16.75,2.5));
#10722=CARTESIAN_POINT('',(5.941847823325,17.16666666667,1.568305009375));
#10723=CARTESIAN_POINT('Ctrl Pts',(5.94184782332521,17.166666666666,1.56830500937566));
#10724=CARTESIAN_POINT('Ctrl Pts',(5.95606809991403,17.2680603300616,1.47761575983942));
#10725=CARTESIAN_POINT('Ctrl Pts',(5.97033187405027,17.3896756931327,1.39989973971076));
#10726=CARTESIAN_POINT('Ctrl Pts',(5.99317707212167,17.6749274551324,1.28155958502111));
#10727=CARTESIAN_POINT('Ctrl Pts',(6.,17.8425551713404,1.25));
#10728=CARTESIAN_POINT('Ctrl Pts',(6.,18.1574448286596,1.25));
#10729=CARTESIAN_POINT('Ctrl Pts',(5.99317707212167,18.3250725448676,1.28155958502111));
#10730=CARTESIAN_POINT('Ctrl Pts',(5.96852269967858,18.6329141822397,1.40927142361291));
#10731=CARTESIAN_POINT('Ctrl Pts',(5.9510289473619,18.7731654856785,1.50539853271216));
#10732=CARTESIAN_POINT('Ctrl Pts',(5.91804743154611,18.9946087962089,1.72684184324257));
#10733=CARTESIAN_POINT('Ctrl Pts',(5.90038488226116,19.0907301683418,1.86709004341607));
#10734=CARTESIAN_POINT('Ctrl Pts',(5.87534197873269,19.2184378409785,2.17492086231842));
#10735=CARTESIAN_POINT('Ctrl Pts',(5.86834729715275,19.25,2.34254474936005));
#10736=CARTESIAN_POINT('Ctrl Pts',(5.86834729715275,19.25,2.5));
#10737=CARTESIAN_POINT('Ctrl Pts',(5.86834729715275,19.25,2.65745525063995));
#10738=CARTESIAN_POINT('Ctrl Pts',(5.87534197873269,19.2184378409785,2.82507913768158));
#10739=CARTESIAN_POINT('Ctrl Pts',(5.90038488226116,19.0907301683418,3.13290995658393));
#10740=CARTESIAN_POINT('Ctrl Pts',(5.91804743154611,18.9946087962089,3.27315815675743));
#10741=CARTESIAN_POINT('Ctrl Pts',(5.9510289473619,18.7731654856785,3.49460146728784));
#10742=CARTESIAN_POINT('Ctrl Pts',(5.96852269967858,18.6329141822397,3.59072857638709));
#10743=CARTESIAN_POINT('Ctrl Pts',(5.99317707212167,18.3250725448676,3.71844041497889));
#10744=CARTESIAN_POINT('Ctrl Pts',(6.,18.1574448286596,3.75));
#10745=CARTESIAN_POINT('Ctrl Pts',(6.,18.,3.75));
#10746=CARTESIAN_POINT('',(5.94184782373737,17.1666666696037,-1.7));
#10747=CARTESIAN_POINT('',(5.941847824424,17.1666666745,-1.7));
#10748=CARTESIAN_POINT('',(-6.,18.,-1.7));
#10749=CARTESIAN_POINT('Origin',(0.,18.,-1.7));
#10750=CARTESIAN_POINT('',(-6.,18.,1.25));
#10751=CARTESIAN_POINT('',(-6.,18.,2.));
#10752=CARTESIAN_POINT('Ctrl Pts',(-6.,18.,3.75));
#10753=CARTESIAN_POINT('Ctrl Pts',(-6.,18.1574448286596,3.75));
#10754=CARTESIAN_POINT('Ctrl Pts',(-5.99317707212167,18.3250725448676,3.71844041497889));
#10755=CARTESIAN_POINT('Ctrl Pts',(-5.96852269967858,18.6329141822397,3.59072857638709));
#10756=CARTESIAN_POINT('Ctrl Pts',(-5.9510289473619,18.7731654856785,3.49460146728784));
#10757=CARTESIAN_POINT('Ctrl Pts',(-5.91804743154611,18.9946087962089,3.27315815675743));
#10758=CARTESIAN_POINT('Ctrl Pts',(-5.90038488226116,19.0907301683418,3.13290995658393));
#10759=CARTESIAN_POINT('Ctrl Pts',(-5.87534197873269,19.2184378409785,2.82507913768158));
#10760=CARTESIAN_POINT('Ctrl Pts',(-5.86834729715275,19.25,2.65745525063995));
#10761=CARTESIAN_POINT('Ctrl Pts',(-5.86834729715275,19.25,2.5));
#10762=CARTESIAN_POINT('Ctrl Pts',(-5.86834729715275,19.25,2.34254474936005));
#10763=CARTESIAN_POINT('Ctrl Pts',(-5.87534197873269,19.2184378409785,2.17492086231842));
#10764=CARTESIAN_POINT('Ctrl Pts',(-5.90038488226116,19.0907301683418,1.86709004341607));
#10765=CARTESIAN_POINT('Ctrl Pts',(-5.91804743154611,18.9946087962089,1.72684184324257));
#10766=CARTESIAN_POINT('Ctrl Pts',(-5.9510289473619,18.7731654856785,1.50539853271216));
#10767=CARTESIAN_POINT('Ctrl Pts',(-5.96852269967858,18.6329141822397,1.40927142361291));
#10768=CARTESIAN_POINT('Ctrl Pts',(-5.99317707212167,18.3250725448676,1.28155958502111));
#10769=CARTESIAN_POINT('Ctrl Pts',(-6.,18.1574448286596,1.25));
#10770=CARTESIAN_POINT('Ctrl Pts',(-6.,18.,1.25));
#10771=CARTESIAN_POINT('Origin',(0.,0.,-2.));
#10772=CARTESIAN_POINT('',(-5.644755432159,17.20833333333,-2.));
#10773=CARTESIAN_POINT('',(5.644755432159,17.20833333333,-2.));
#10774=CARTESIAN_POINT('Origin',(0.,18.,-2.));
#10775=CARTESIAN_POINT('',(3.168985505772,-0.4444444444442,-2.));
#10776=CARTESIAN_POINT('',(5.644755432159,17.20833333333,-2.));
#10777=CARTESIAN_POINT('',(-3.168985505773,-0.4444444444444,-2.));
#10778=CARTESIAN_POINT('Origin',(0.,0.,-2.));
#10779=CARTESIAN_POINT('',(-3.168985505773,-0.4444444444444,-2.));
#10780=CARTESIAN_POINT('',(-2.5,18.,-2.));
#10781=CARTESIAN_POINT('Origin',(0.,18.,-2.));
#10782=CARTESIAN_POINT('',(-1.25,-1.53080849893419E-16,-2.));
#10783=CARTESIAN_POINT('Origin',(0.,0.,-2.));
#10784=CARTESIAN_POINT('Origin',(0.,0.,-2.));
#10785=CARTESIAN_POINT('',(-1.25,-1.53080849893419E-16,2.));
#10786=CARTESIAN_POINT('',(-1.25,-1.53080849893419E-16,-2.));
#10787=CARTESIAN_POINT('Origin',(0.,0.,2.));
#10788=CARTESIAN_POINT('Origin',(0.,0.,2.));
#10789=CARTESIAN_POINT('',(-5.594625601103,14.69089674028,2.));
#10790=CARTESIAN_POINT('',(5.594625601103,14.69089674028,2.));
#10791=CARTESIAN_POINT('Origin',(0.,18.,2.));
#10792=CARTESIAN_POINT('',(-3.46607789694,-0.4861111111111,2.));
#10793=CARTESIAN_POINT('',(-5.594625601103,14.69089674028,2.));
#10794=CARTESIAN_POINT('',(3.46607789694,-0.4861111111111,2.));
#10795=CARTESIAN_POINT('Origin',(0.,0.,2.));
#10796=CARTESIAN_POINT('',(3.46607789694,-0.4861111111111,2.));
#10797=CARTESIAN_POINT('Origin',(0.,18.,2.5));
#10798=CARTESIAN_POINT('',(5.884205625306,16.75566526407,2.38112584404));
#10799=CARTESIAN_POINT('Ctrl Pts',(5.88420562530688,16.7556652640704,2.38112584403824));
#10800=CARTESIAN_POINT('Ctrl Pts',(5.79043247403846,16.0870423103697,2.19077963448577));
#10801=CARTESIAN_POINT('Ctrl Pts',(5.68686691397717,15.3485973532238,2.));
#10802=CARTESIAN_POINT('Ctrl Pts',(5.59462560110366,14.6908967402821,2.));
#10803=CARTESIAN_POINT('Ctrl Pts',(5.86834729715275,16.75,2.5));
#10804=CARTESIAN_POINT('Ctrl Pts',(5.86834729715275,16.75,2.48193013436365));
#10805=CARTESIAN_POINT('Ctrl Pts',(5.86943196932979,16.7503925868786,2.46381885206853));
#10806=CARTESIAN_POINT('Ctrl Pts',(5.87426960134035,16.7521318837435,2.42379416578773));
#10807=CARTESIAN_POINT('Ctrl Pts',(5.87850100129599,16.7536496858429,2.40222423989646));
#10808=CARTESIAN_POINT('Ctrl Pts',(5.88420562530614,16.7556652640689,2.38112584403993));
#10809=CARTESIAN_POINT('',(-5.884205625306,16.75566526407,2.38112584404));
#10810=CARTESIAN_POINT('Ctrl Pts',(-5.88420562530614,16.7556652640689,2.38112584403993));
#10811=CARTESIAN_POINT('Ctrl Pts',(-5.88352496284375,16.7554247699651,2.38364325553814));
#10812=CARTESIAN_POINT('Ctrl Pts',(-5.88286503903123,16.7551912573634,2.38616828635534));
#10813=CARTESIAN_POINT('Ctrl Pts',(-5.87300883084945,16.7516991206043,2.42523264769952));
#10814=CARTESIAN_POINT('Ctrl Pts',(-5.86834729715275,16.75,2.46252726842572));
#10815=CARTESIAN_POINT('Ctrl Pts',(-5.86834729715275,16.75,2.5));
#10816=CARTESIAN_POINT('Ctrl Pts',(-5.59462560110203,14.6908967402794,2.));
#10817=CARTESIAN_POINT('Ctrl Pts',(-5.68686691397567,15.348597353222,2.00000000000015));
#10818=CARTESIAN_POINT('Ctrl Pts',(-5.79043247403725,16.0870423103699,2.19077963448226));
#10819=CARTESIAN_POINT('Ctrl Pts',(-5.88420562530548,16.7556652640693,2.3811258440429));
#10820=CARTESIAN_POINT('Origin',(-5.941847823325,17.16666666667,-2.));
#10821=CARTESIAN_POINT('',(-3.46607789546553,-0.48611112162235,-1.7));
#10822=CARTESIAN_POINT('',(-5.94184782319004,17.1666666657008,-1.7));
#10823=CARTESIAN_POINT('',(-3.466077893795,-0.4861111335351,-1.7));
#10824=CARTESIAN_POINT('',(-3.466077893795,-0.4861111335351,-1.7));
#10825=CARTESIAN_POINT('',(-5.941847823325,17.16666666667,1.568305009375));
#10826=CARTESIAN_POINT('Origin',(-6.05872130529396,18.,2.5));
#10827=CARTESIAN_POINT('',(-5.941847822783,17.1666666628,-1.7));
#10828=CARTESIAN_POINT('Origin',(-3.13864717244,-0.6607633563004,-1.7));
#10829=CARTESIAN_POINT('Origin',(-3.168985505773,-0.4444444444444,-1.7));
#10830=CARTESIAN_POINT('Origin',(-5.644755432159,17.20833333333,-1.7));
#10831=CARTESIAN_POINT('Origin',(0.,18.,-1.7));
#10832=CARTESIAN_POINT('Origin',(0.,18.,-1.7));
#10833=CARTESIAN_POINT('Origin',(5.644755432159,17.20833333333,-1.7));
#10834=CARTESIAN_POINT('Origin',(5.675093765492,17.42465224519,-1.7));
#10835=CARTESIAN_POINT('',(3.46607789817656,-0.486111102291924,-1.7));
#10836=CARTESIAN_POINT('',(5.941847824424,17.1666666745,-1.7));
#10837=CARTESIAN_POINT('Origin',(3.168985505773,-0.4444444444444,-1.7));
#10838=CARTESIAN_POINT('Origin',(0.,0.,-1.7));
#10839=CARTESIAN_POINT('Origin',(0.,0.,-1.7));
#10840=CARTESIAN_POINT('Origin',(0.,0.,-2.));
#10841=CARTESIAN_POINT('',(3.466077899139,-0.4861110954326,-1.7));
#10842=CARTESIAN_POINT('Origin',(3.46607789694,-0.4861111111111,-2.));
#10843=CARTESIAN_POINT('Origin',(6.05872130529521,18.,2.5));
#10844=CARTESIAN_POINT('Origin',(-7.75,18.,2.5));
#10845=CARTESIAN_POINT('Ctrl Pts',(-6.,18.,1.25));
#10846=CARTESIAN_POINT('Ctrl Pts',(-6.,17.8425551713404,1.25));
#10847=CARTESIAN_POINT('Ctrl Pts',(-5.99317707212167,17.6749274551324,1.28155958502111));
#10848=CARTESIAN_POINT('Ctrl Pts',(-5.97033187405036,17.3896756931338,1.39989973971032));
#10849=CARTESIAN_POINT('Ctrl Pts',(-5.95606809991427,17.2680603300636,1.47761575983813));
#10850=CARTESIAN_POINT('Ctrl Pts',(-5.94184782332556,17.1666666666685,1.56830500937343));
#10851=CARTESIAN_POINT('',(-2.5,18.,3.75));
#10852=CARTESIAN_POINT('',(-7.75,18.,3.75));
#10853=CARTESIAN_POINT('',(-2.5,18.,1.25));
#10854=CARTESIAN_POINT('Ctrl Pts',(-2.5,18.,1.25));
#10855=CARTESIAN_POINT('Ctrl Pts',(-2.5,17.8400558736141,1.25));
#10856=CARTESIAN_POINT('Ctrl Pts',(-2.48323996043832,17.6713186556389,1.28254511766359));
#10857=CARTESIAN_POINT('Ctrl Pts',(-2.42283105129935,17.364074052357,1.41104365009428));
#10858=CARTESIAN_POINT('Ctrl Pts',(-2.37983326258812,17.2253791627422,1.50685388429146));
#10859=CARTESIAN_POINT('Ctrl Pts',(-2.29712558443605,17.0065552148362,1.72567783219742));
#10860=CARTESIAN_POINT('Ctrl Pts',(-2.25149501557585,16.9109641128297,1.86427205061522));
#10861=CARTESIAN_POINT('Ctrl Pts',(-2.18478179494117,16.7826430194041,2.17107674842089));
#10862=CARTESIAN_POINT('Ctrl Pts',(-2.1650635094611,16.75,2.33961866629939));
#10863=CARTESIAN_POINT('Ctrl Pts',(-2.1650635094611,16.75,2.66038133370061));
#10864=CARTESIAN_POINT('Ctrl Pts',(-2.18478179494117,16.7826430194041,2.82892325157911));
#10865=CARTESIAN_POINT('Ctrl Pts',(-2.25149501557585,16.9109641128297,3.13572794938478));
#10866=CARTESIAN_POINT('Ctrl Pts',(-2.29712558443605,17.0065552148362,3.27432216780258));
#10867=CARTESIAN_POINT('Ctrl Pts',(-2.37983326258812,17.2253791627422,3.49314611570854));
#10868=CARTESIAN_POINT('Ctrl Pts',(-2.42283105129935,17.364074052357,3.58895634990573));
#10869=CARTESIAN_POINT('Ctrl Pts',(-2.48323996043832,17.6713186556389,3.71745488233641));
#10870=CARTESIAN_POINT('Ctrl Pts',(-2.5,17.8400558736141,3.75));
#10871=CARTESIAN_POINT('Ctrl Pts',(-2.5,18.,3.75));
#10872=CARTESIAN_POINT('Ctrl Pts',(-2.5,18.,3.75));
#10873=CARTESIAN_POINT('Ctrl Pts',(-2.5,18.1599441263859,3.75));
#10874=CARTESIAN_POINT('Ctrl Pts',(-2.48323996043832,18.3286813443611,3.71745488233641));
#10875=CARTESIAN_POINT('Ctrl Pts',(-2.42283105129935,18.635925947643,3.58895634990573));
#10876=CARTESIAN_POINT('Ctrl Pts',(-2.37983326258812,18.7746208372578,3.49314611570854));
#10877=CARTESIAN_POINT('Ctrl Pts',(-2.29712558443605,18.9934447851638,3.27432216780258));
#10878=CARTESIAN_POINT('Ctrl Pts',(-2.25149501557585,19.0890358871703,3.13572794938478));
#10879=CARTESIAN_POINT('Ctrl Pts',(-2.18478179494117,19.2173569805959,2.82892325157911));
#10880=CARTESIAN_POINT('Ctrl Pts',(-2.1650635094611,19.25,2.66038133370061));
#10881=CARTESIAN_POINT('Ctrl Pts',(-2.1650635094611,19.25,2.5));
#10882=CARTESIAN_POINT('Ctrl Pts',(-2.1650635094611,19.25,2.33961866629939));
#10883=CARTESIAN_POINT('Ctrl Pts',(-2.18478179494117,19.2173569805959,2.17107674842089));
#10884=CARTESIAN_POINT('Ctrl Pts',(-2.25149501557585,19.0890358871703,1.86427205061522));
#10885=CARTESIAN_POINT('Ctrl Pts',(-2.29712558443605,18.9934447851638,1.72567783219742));
#10886=CARTESIAN_POINT('Ctrl Pts',(-2.37983326258812,18.7746208372578,1.50685388429146));
#10887=CARTESIAN_POINT('Ctrl Pts',(-2.42283105129935,18.635925947643,1.41104365009428));
#10888=CARTESIAN_POINT('Ctrl Pts',(-2.48323996043832,18.3286813443611,1.28254511766359));
#10889=CARTESIAN_POINT('Ctrl Pts',(-2.5,18.1599441263859,1.25));
#10890=CARTESIAN_POINT('Ctrl Pts',(-2.5,18.,1.25));
#10891=CARTESIAN_POINT('Origin',(-7.75,18.,2.5));
#10892=CARTESIAN_POINT('',(2.5,18.,1.25));
#10893=CARTESIAN_POINT('',(2.5,18.,3.75));
#10894=CARTESIAN_POINT('Ctrl Pts',(2.5,18.,1.25));
#10895=CARTESIAN_POINT('Ctrl Pts',(2.5,18.1599441263859,1.25));
#10896=CARTESIAN_POINT('Ctrl Pts',(2.48323996043832,18.3286813443611,1.28254511766359));
#10897=CARTESIAN_POINT('Ctrl Pts',(2.42283105129935,18.635925947643,1.41104365009428));
#10898=CARTESIAN_POINT('Ctrl Pts',(2.37983326258812,18.7746208372578,1.50685388429146));
#10899=CARTESIAN_POINT('Ctrl Pts',(2.29712558443605,18.9934447851638,1.72567783219742));
#10900=CARTESIAN_POINT('Ctrl Pts',(2.25149501557585,19.0890358871703,1.86427205061522));
#10901=CARTESIAN_POINT('Ctrl Pts',(2.18478179494117,19.2173569805959,2.17107674842089));
#10902=CARTESIAN_POINT('Ctrl Pts',(2.1650635094611,19.25,2.33961866629939));
#10903=CARTESIAN_POINT('Ctrl Pts',(2.1650635094611,19.25,2.5));
#10904=CARTESIAN_POINT('Ctrl Pts',(2.1650635094611,19.25,2.66038133370061));
#10905=CARTESIAN_POINT('Ctrl Pts',(2.18478179494117,19.2173569805959,2.82892325157911));
#10906=CARTESIAN_POINT('Ctrl Pts',(2.25149501557585,19.0890358871703,3.13572794938478));
#10907=CARTESIAN_POINT('Ctrl Pts',(2.29712558443605,18.9934447851638,3.27432216780258));
#10908=CARTESIAN_POINT('Ctrl Pts',(2.37983326258812,18.7746208372578,3.49314611570854));
#10909=CARTESIAN_POINT('Ctrl Pts',(2.42283105129935,18.635925947643,3.58895634990573));
#10910=CARTESIAN_POINT('Ctrl Pts',(2.48323996043832,18.3286813443611,3.71745488233641));
#10911=CARTESIAN_POINT('Ctrl Pts',(2.5,18.1599441263859,3.75));
#10912=CARTESIAN_POINT('Ctrl Pts',(2.5,18.,3.75));
#10913=CARTESIAN_POINT('Ctrl Pts',(2.5,18.,3.75));
#10914=CARTESIAN_POINT('Ctrl Pts',(2.5,17.8400558736141,3.75));
#10915=CARTESIAN_POINT('Ctrl Pts',(2.48323996043832,17.6713186556389,3.71745488233641));
#10916=CARTESIAN_POINT('Ctrl Pts',(2.42283105129935,17.364074052357,3.58895634990573));
#10917=CARTESIAN_POINT('Ctrl Pts',(2.37983326258812,17.2253791627422,3.49314611570854));
#10918=CARTESIAN_POINT('Ctrl Pts',(2.29712558443605,17.0065552148362,3.27432216780258));
#10919=CARTESIAN_POINT('Ctrl Pts',(2.25149501557585,16.9109641128297,3.13572794938478));
#10920=CARTESIAN_POINT('Ctrl Pts',(2.18478179494117,16.7826430194041,2.82892325157911));
#10921=CARTESIAN_POINT('Ctrl Pts',(2.1650635094611,16.75,2.66038133370061));
#10922=CARTESIAN_POINT('Ctrl Pts',(2.1650635094611,16.75,2.33961866629939));
#10923=CARTESIAN_POINT('Ctrl Pts',(2.18478179494117,16.7826430194041,2.17107674842089));
#10924=CARTESIAN_POINT('Ctrl Pts',(2.25149501557585,16.9109641128297,1.86427205061523));
#10925=CARTESIAN_POINT('Ctrl Pts',(2.29712558443605,17.0065552148362,1.72567783219742));
#10926=CARTESIAN_POINT('Ctrl Pts',(2.37983326258812,17.2253791627422,1.50685388429146));
#10927=CARTESIAN_POINT('Ctrl Pts',(2.42283105129935,17.364074052357,1.41104365009428));
#10928=CARTESIAN_POINT('Ctrl Pts',(2.48323996043832,17.6713186556389,1.28254511766359));
#10929=CARTESIAN_POINT('Ctrl Pts',(2.5,17.8400558736141,1.25));
#10930=CARTESIAN_POINT('Ctrl Pts',(2.5,18.,1.25));
#10931=CARTESIAN_POINT('',(-7.75,18.,3.75));
#10932=CARTESIAN_POINT('Origin',(0.,18.,2.));
#10933=CARTESIAN_POINT('Origin',(0.,18.,-2.));
#10934=CARTESIAN_POINT('',(-2.5,18.,-2.));
#10935=CARTESIAN_POINT('',(-2.5,18.,5.));
#10936=CARTESIAN_POINT('',(-2.5,18.,-2.));
#10937=CARTESIAN_POINT('Origin',(0.,18.,5.));
#10938=CARTESIAN_POINT('Origin',(0.,0.,5.));
#10939=CARTESIAN_POINT('Origin',(0.,0.,2.));
#10940=CARTESIAN_POINT('',(-1.5,-1.83697019872103E-16,2.));
#10941=CARTESIAN_POINT('Origin',(0.,0.,2.));
#10942=CARTESIAN_POINT('',(-1.5,-1.83697019872103E-16,-2.));
#10943=CARTESIAN_POINT('',(-1.5,-1.83697019872103E-16,2.));
#10944=CARTESIAN_POINT('Origin',(0.,0.,-2.));
#10945=CARTESIAN_POINT('Origin',(0.,0.,-2.));
#10946=CARTESIAN_POINT('',(1.25,0.,-2.));
#10947=CARTESIAN_POINT('Origin',(0.,0.,-2.));
#17077=UNCERTAINTY_MEASURE_WITH_UNIT(LENGTH_MEASURE(0.01),#17114,
'DISTANCE_ACCURACY_VALUE',
'Maximum model space distance between geometric entities at asserted c
onnectivities');
#17090=UNCERTAINTY_MEASURE_WITH_UNIT(LENGTH_MEASURE(0.01),#17114,
'DISTANCE_ACCURACY_VALUE',
'Maximum model space distance between geometric entities at asserted c
onnectivities');
#17100=(
GEOMETRIC_REPRESENTATION_CONTEXT(3)
GLOBAL_UNCERTAINTY_ASSIGNED_CONTEXT((#17077))
GLOBAL_UNIT_ASSIGNED_CONTEXT((#17114,#17116,#17117))
REPRESENTATION_CONTEXT('','3D')
);
#17113=(
GEOMETRIC_REPRESENTATION_CONTEXT(3)
GLOBAL_UNCERTAINTY_ASSIGNED_CONTEXT((#17090))
GLOBAL_UNIT_ASSIGNED_CONTEXT((#17114,#17116,#17117))
REPRESENTATION_CONTEXT('','3D')
);
#17114=(
LENGTH_UNIT()
NAMED_UNIT(*)
SI_UNIT(.MILLI.,.METRE.)
);
#17116=(
NAMED_UNIT(*)
PLANE_ANGLE_UNIT()
SI_UNIT($,.RADIAN.)
);
#17117=(
NAMED_UNIT(*)
SI_UNIT($,.STERADIAN.)
SOLID_ANGLE_UNIT()
);
#17127=SHAPE_DEFINITION_REPRESENTATION(#17153,#17193);
#17153=PRODUCT_DEFINITION_SHAPE('',$,#17216);
#17193=SHAPE_REPRESENTATION('',(#6610,#245),#17100);
#17206=PRODUCT_DEFINITION_CONTEXT('part definition',#17274,'design');
#17216=PRODUCT_DEFINITION('7-2','7-2',#17238,#17206);
#17238=PRODUCT_DEFINITION_FORMATION('',$,#17285);
#17274=APPLICATION_CONTEXT(
'Core Data for Automotive Mechanical Design Process');
#17275=PRODUCT_CONTEXT('part definition',#17274,'mechanical');
#17285=PRODUCT('7-2','7-2','NOT SPECIFIED',(#17275));
#17298=PRESENTATION_STYLE_ASSIGNMENT((#17299));
#17299=SURFACE_STYLE_USAGE(.BOTH.,#17300);
#17300=SURFACE_SIDE_STYLE('',(#17301));
#17301=SURFACE_STYLE_FILL_AREA(#17302);
#17302=FILL_AREA_STYLE('Steel - Satin',(#17303));
#17303=FILL_AREA_STYLE_COLOUR('Steel - Satin',#17304);
#17304=COLOUR_RGB('Steel - Satin', 0.09019608, 0.27058824, 0.51372549);
ENDSEC;
END-ISO-10303-21;
